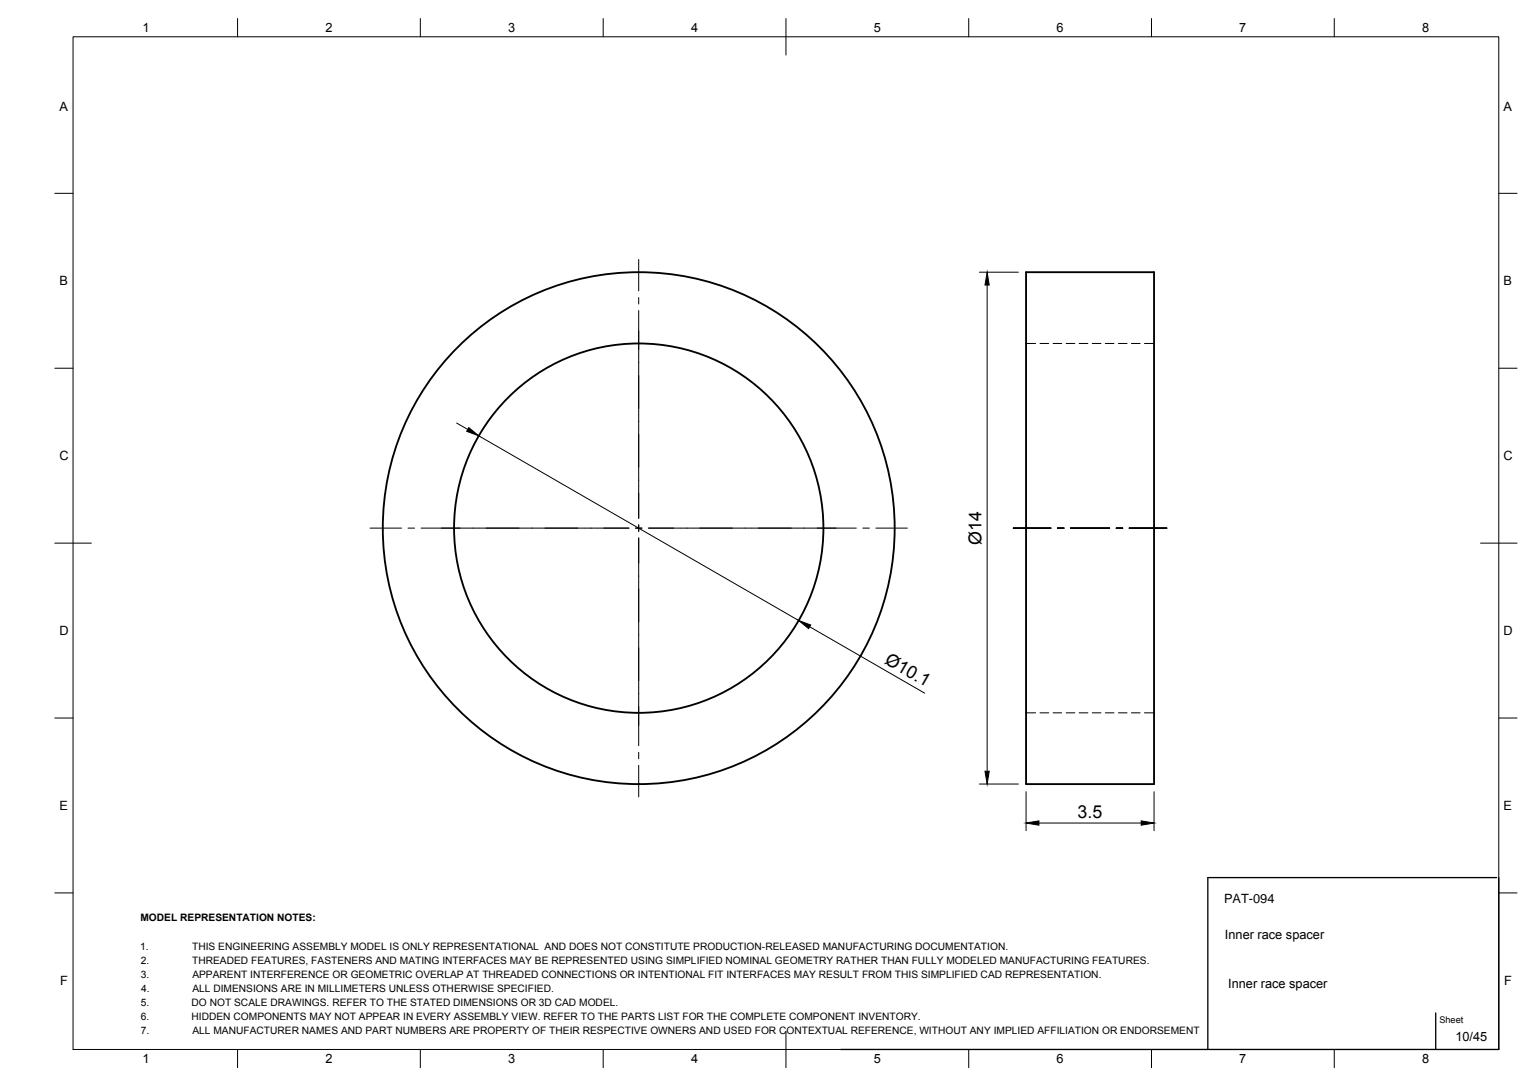
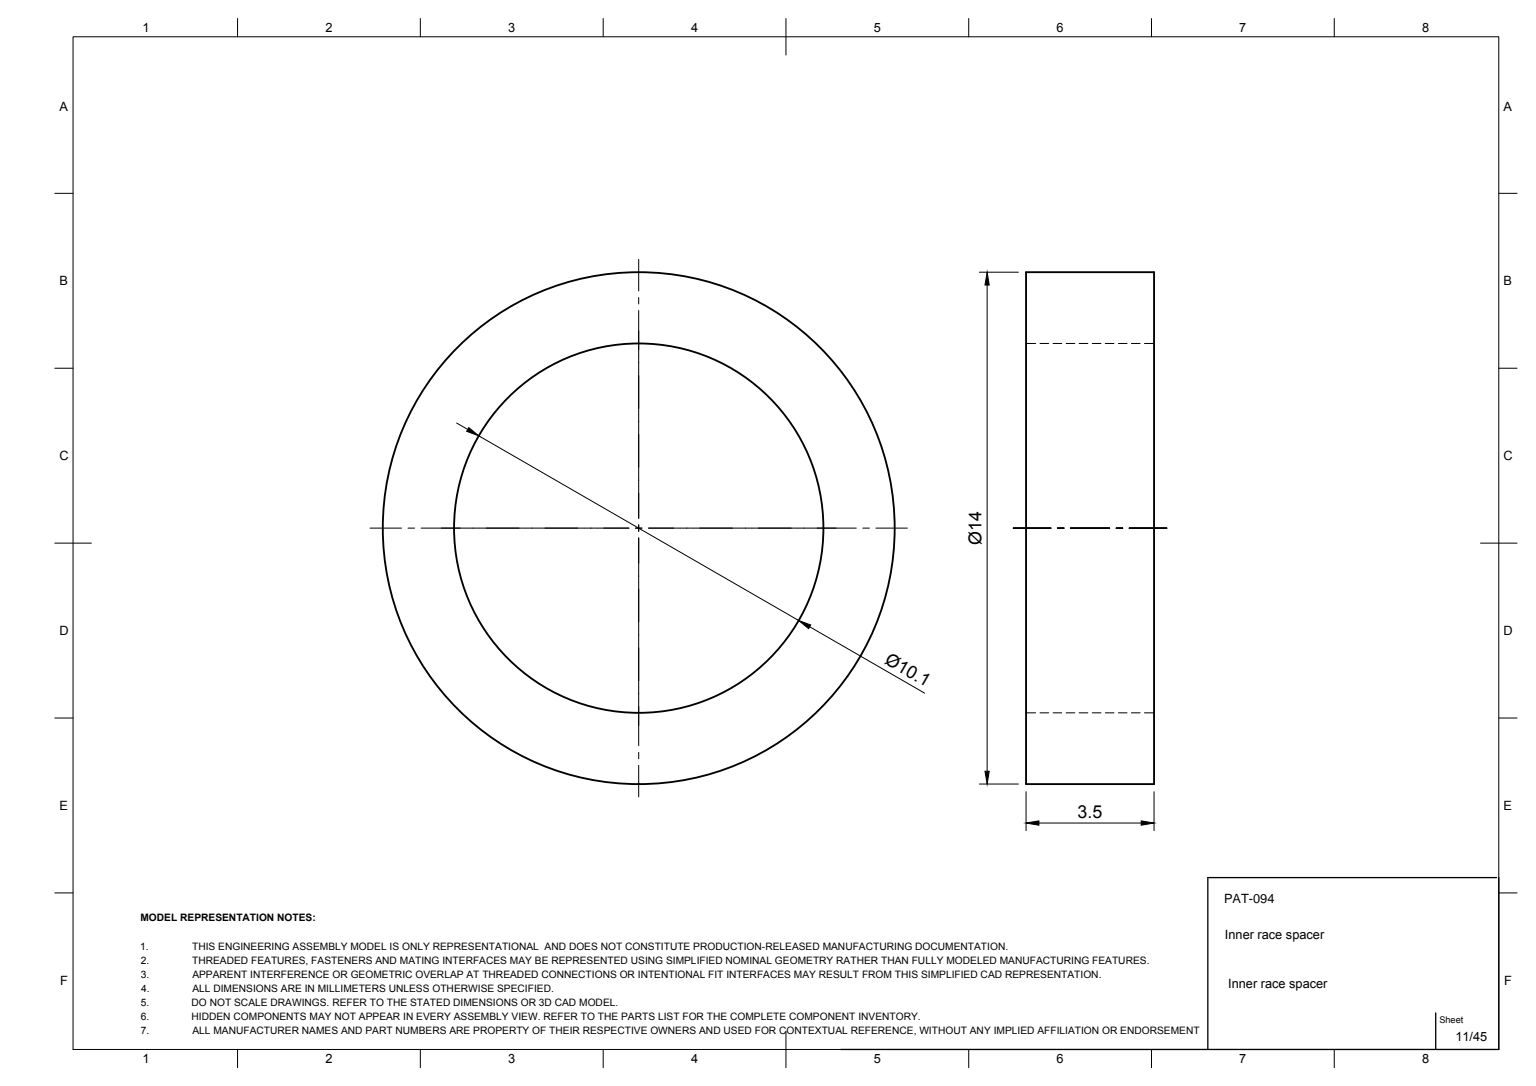
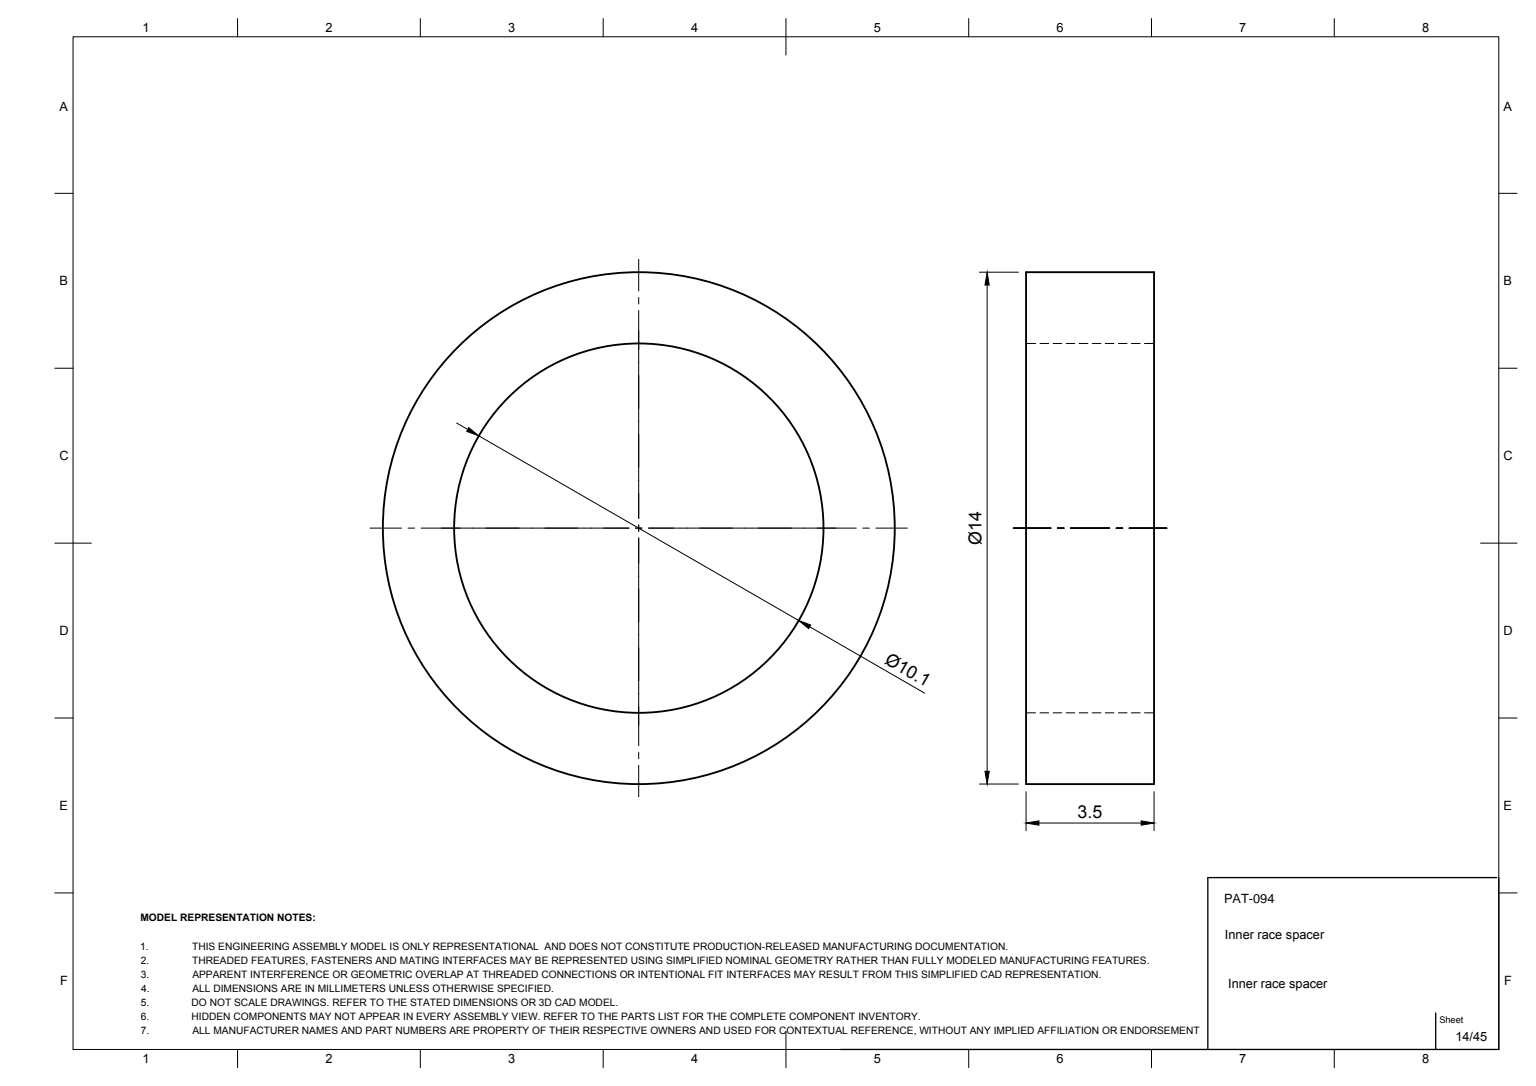
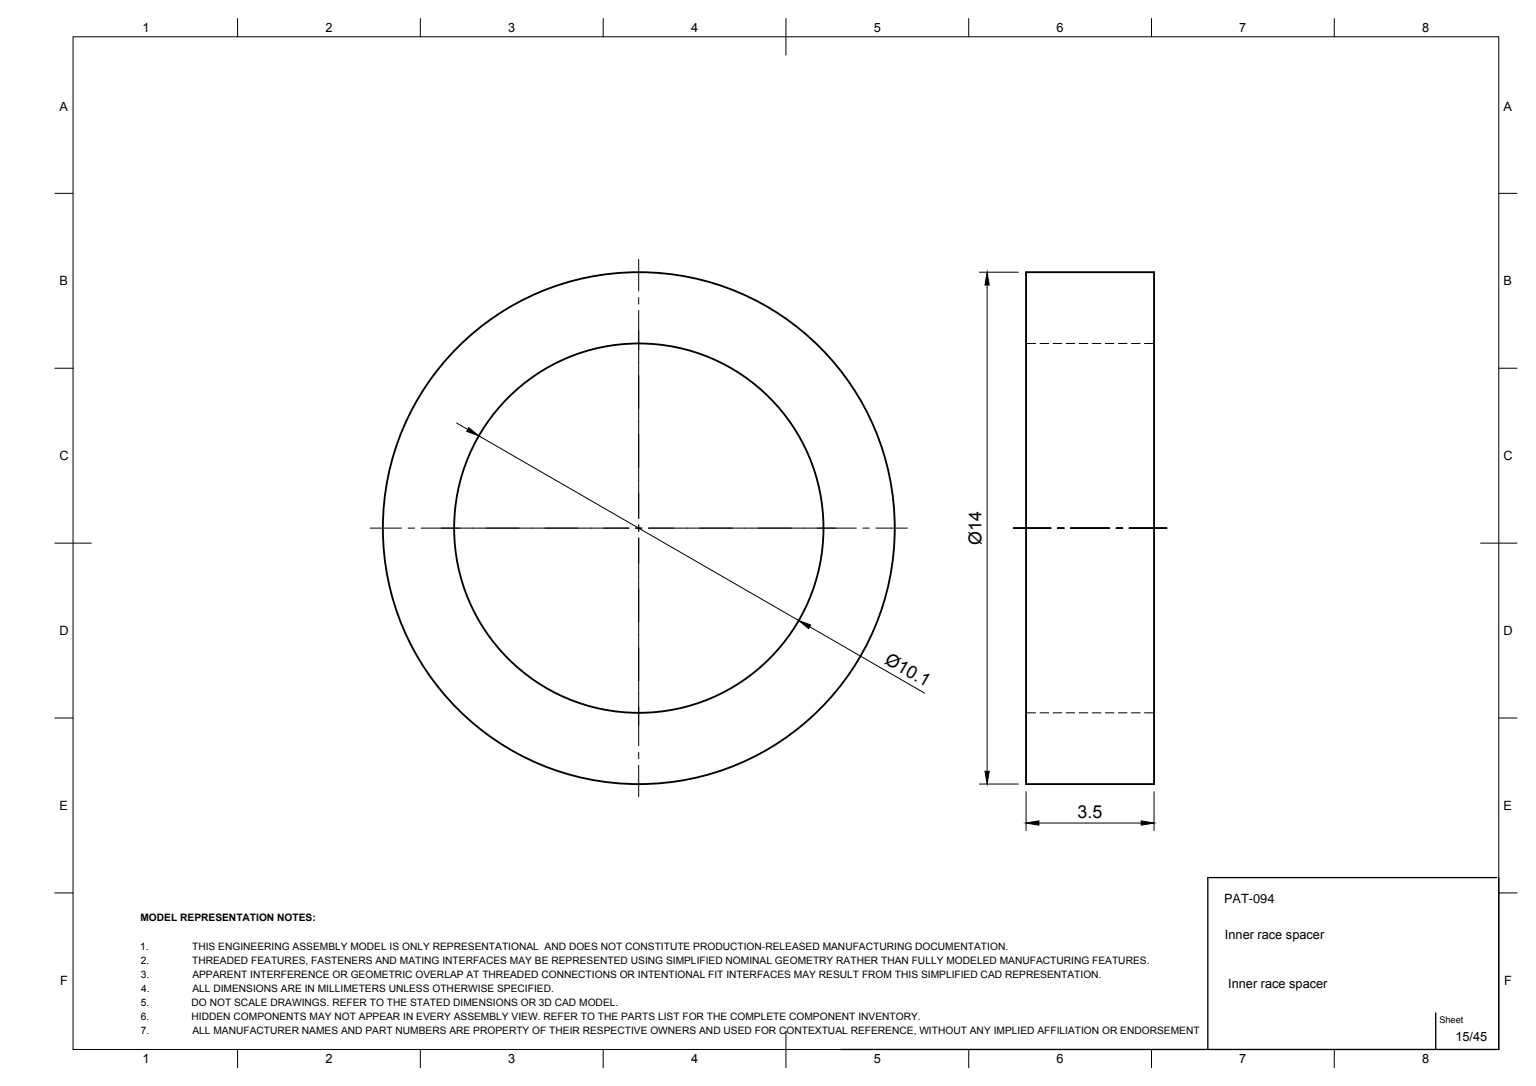
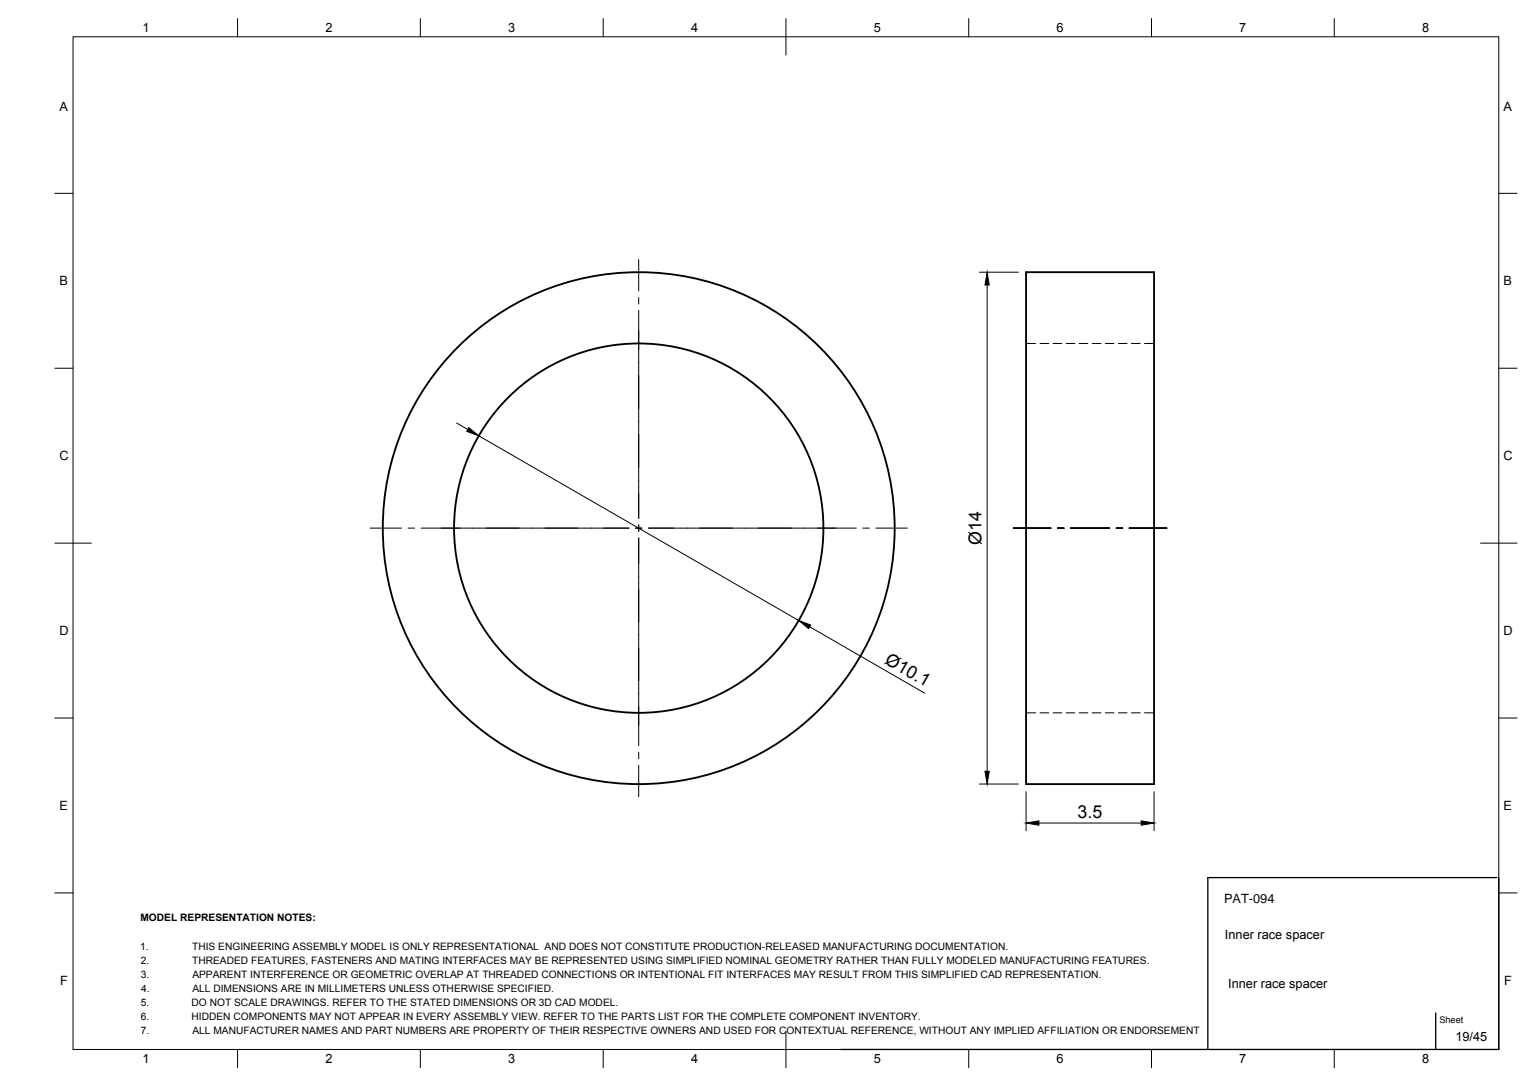
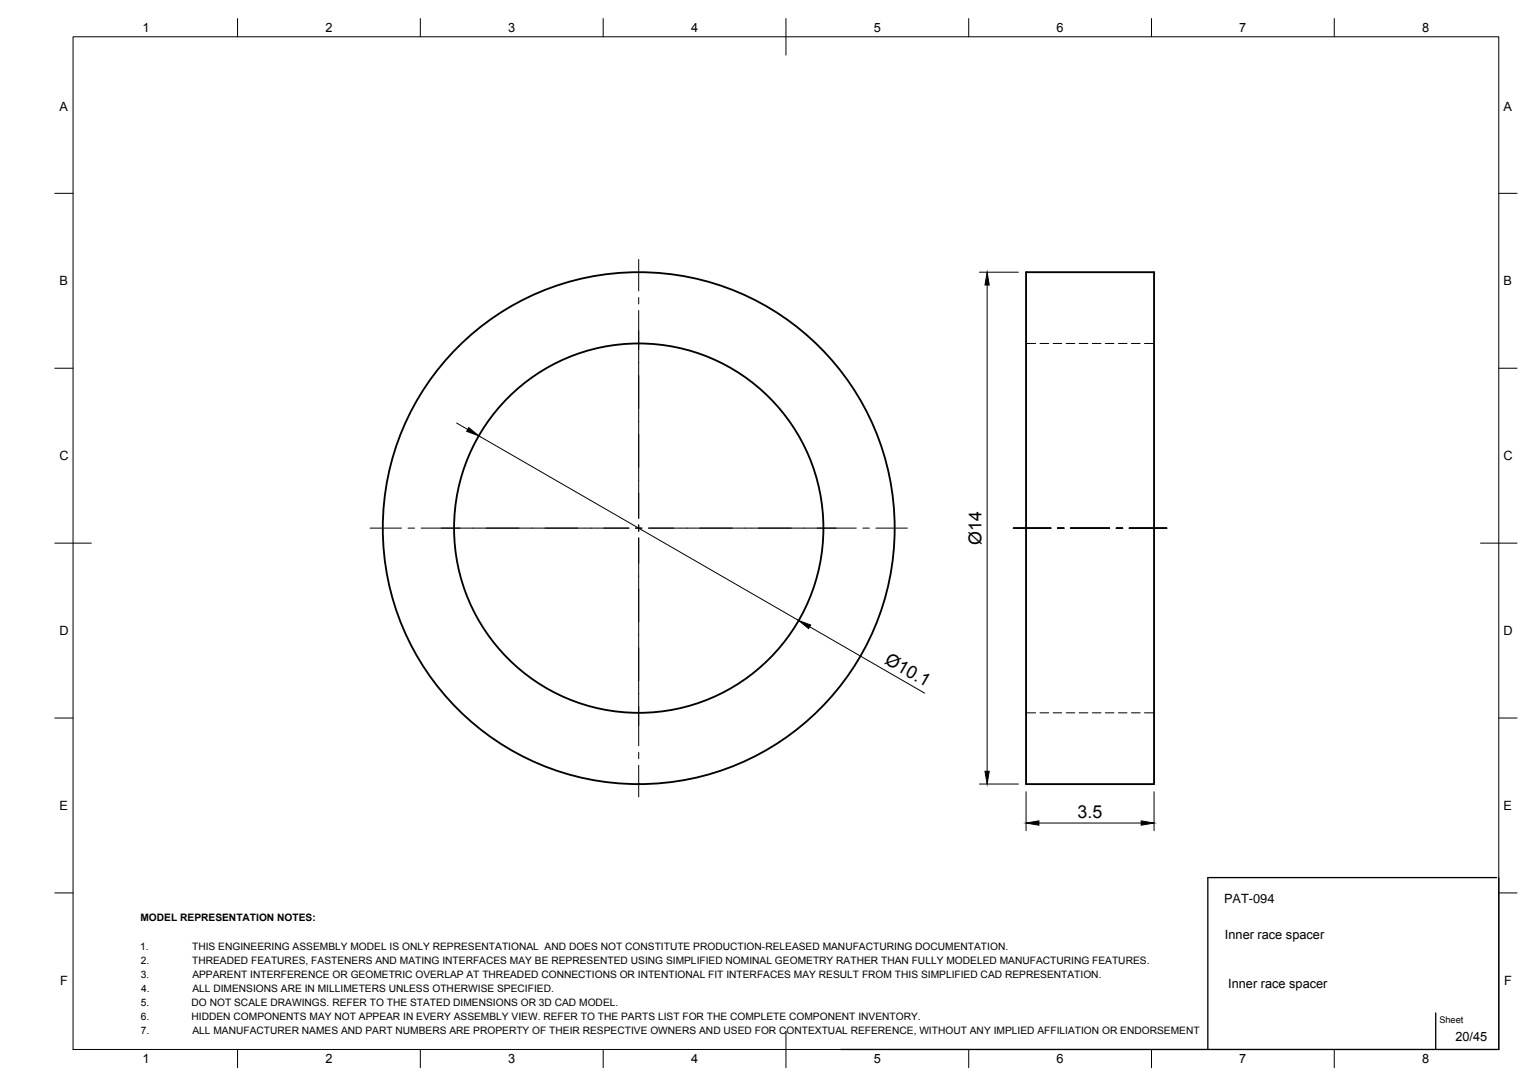
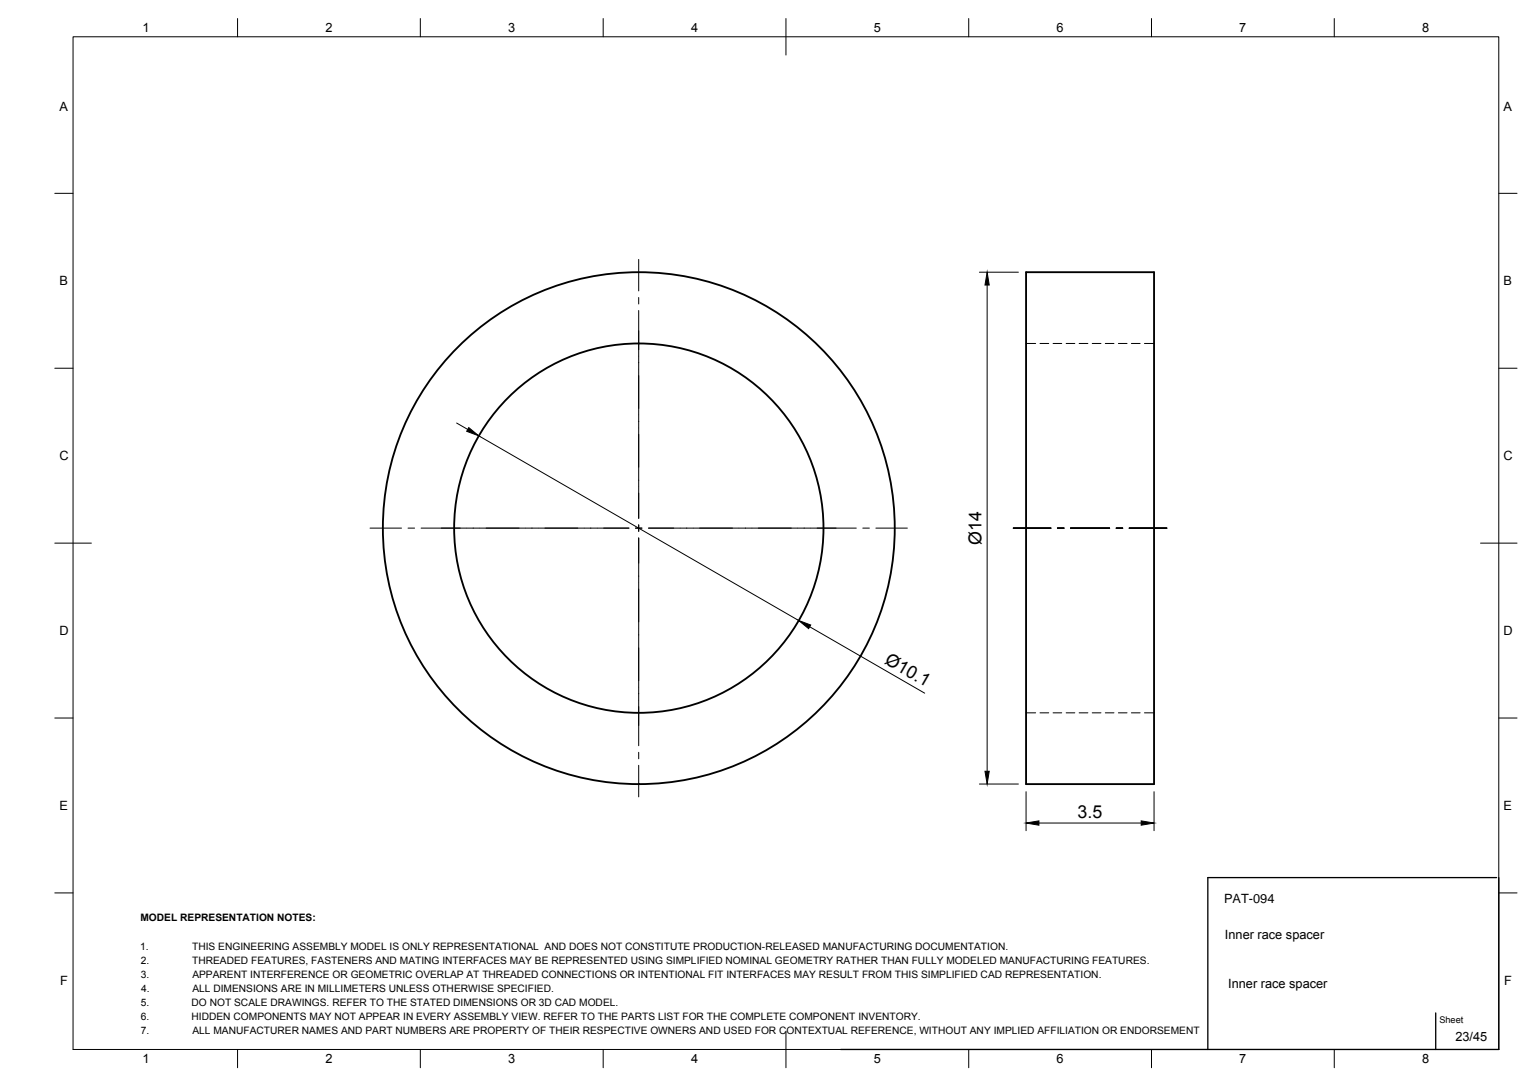
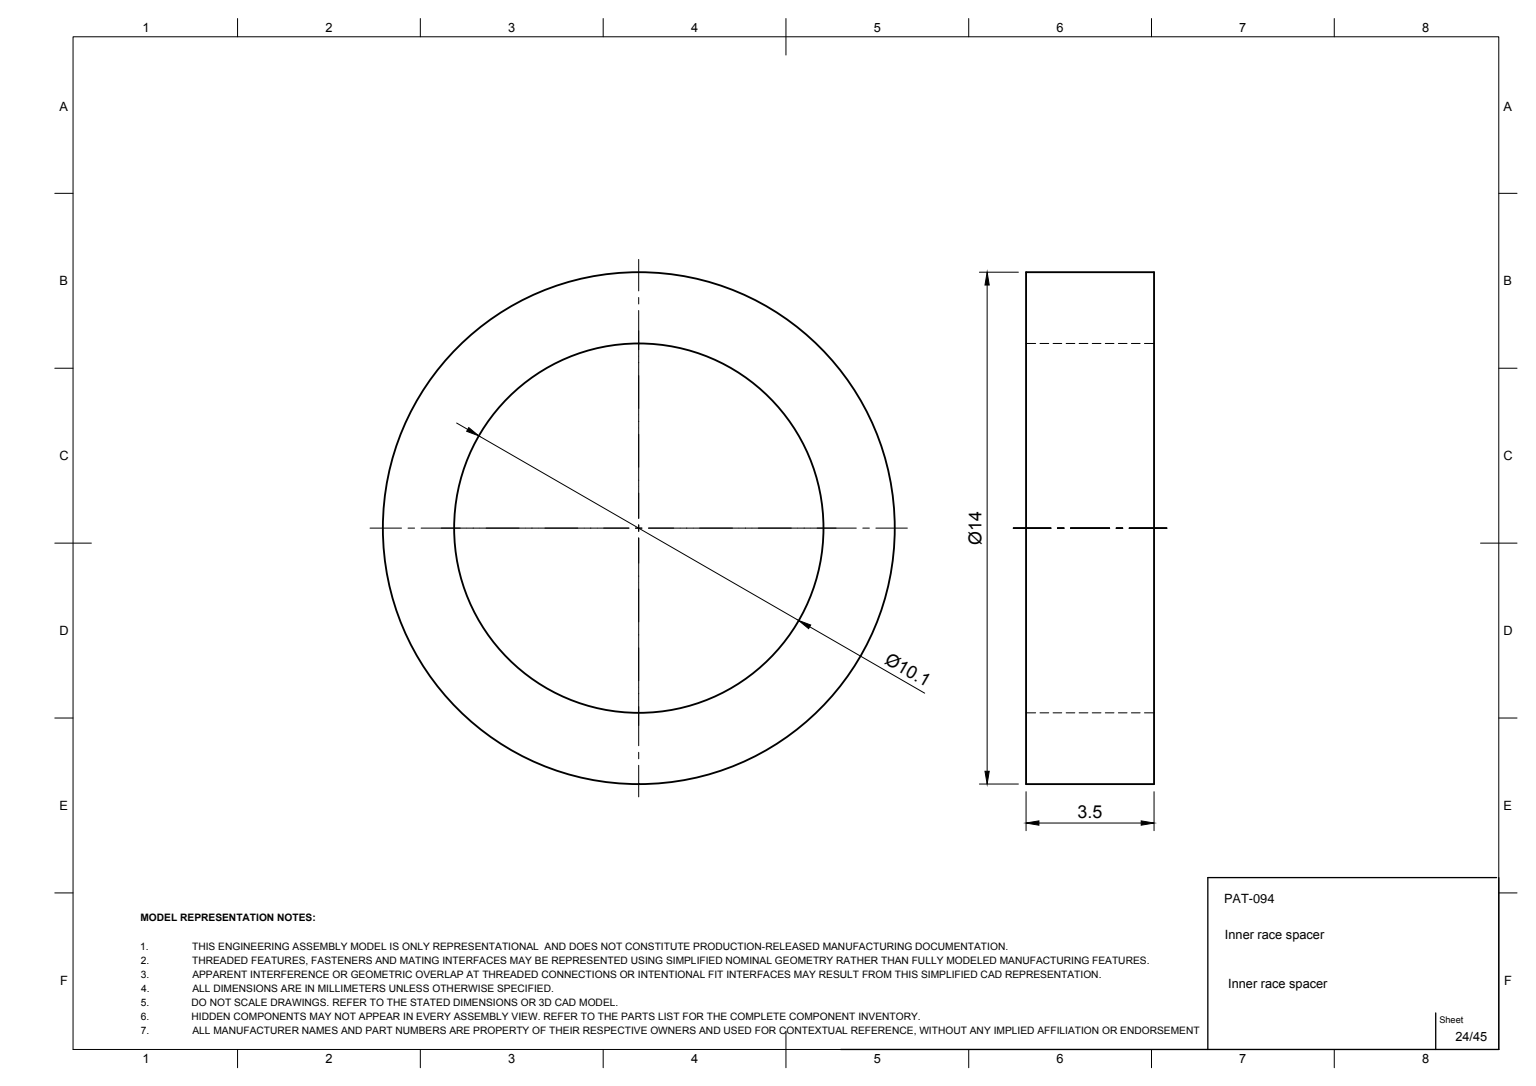
ISO-10303-21;
HEADER;
/* Generated by software containing ST-Developer
 * from STEP Tools, Inc. (www.steptools.com) 
 */

FILE_DESCRIPTION(
/* description */ ('Shaft runout checking stand'),
/* implementation_level */ '2;1');

FILE_NAME(
/* name */ 'Inner race spacer.step',
/* time_stamp */ '2026-11-02T21:12:33-08:00',
/* author */ (''),
/* organization */ (''),
/* preprocessor_version */ 'ST-DEVELOPER v20.2',
/* originating_system */ 'Autodesk Translation Framework v15.17.0.0',
/* authorisation */ '');

FILE_SCHEMA (('AUTOMOTIVE_DESIGN { 1 0 10303 214 3 1 1 }'));
ENDSEC;

DATA;
#10=MECHANICAL_DESIGN_GEOMETRIC_PRESENTATION_REPRESENTATION('',(#471),#11748);
#385=SHAPE_REPRESENTATION_RELATIONSHIP('SRR','None',#11934,#428);
#428=ADVANCED_BREP_SHAPE_REPRESENTATION('',(#522),#11710);
#471=STYLED_ITEM('',(#12170),#522);
#522=MANIFOLD_SOLID_BREP('Body1',#6214);
#601=FACE_BOUND('',#1565,.T.);
#602=FACE_BOUND('',#1567,.T.);
#724=CIRCLE('',#6916,0.505);
#725=CIRCLE('',#6917,0.505);
#726=CIRCLE('',#6919,0.7);
#727=CIRCLE('',#6920,0.7);
#962=CYLINDRICAL_SURFACE('',#6915,0.505);
#963=CYLINDRICAL_SURFACE('',#6918,0.7);
#1155=FACE_OUTER_BOUND('',#1562,.T.);
#1156=FACE_OUTER_BOUND('',#1563,.T.);
#1157=FACE_OUTER_BOUND('',#1564,.T.);
#1158=FACE_OUTER_BOUND('',#1566,.T.);
#1562=EDGE_LOOP('',(#4686,#4687,#4688,#4689));
#1563=EDGE_LOOP('',(#4690,#4691,#4692,#4693));
#1564=EDGE_LOOP('',(#4694));
#1565=EDGE_LOOP('',(#4695));
#1566=EDGE_LOOP('',(#4696));
#1567=EDGE_LOOP('',(#4697));
#2131=LINE('',#10105,#2598);
#2132=LINE('',#10111,#2599);
#2598=VECTOR('',#8104,0.505);
#2599=VECTOR('',#8111,0.7);
#3018=VERTEX_POINT('',#10102);
#3019=VERTEX_POINT('',#10104);
#3020=VERTEX_POINT('',#10108);
#3021=VERTEX_POINT('',#10110);
#3629=EDGE_CURVE('',#3018,#3018,#724,.T.);
#3630=EDGE_CURVE('',#3018,#3019,#2131,.T.);
#3631=EDGE_CURVE('',#3019,#3019,#725,.T.);
#3632=EDGE_CURVE('',#3020,#3020,#726,.T.);
#3633=EDGE_CURVE('',#3020,#3021,#2132,.T.);
#3634=EDGE_CURVE('',#3021,#3021,#727,.T.);
#4686=ORIENTED_EDGE('',*,*,#3629,.F.);
#4687=ORIENTED_EDGE('',*,*,#3630,.T.);
#4688=ORIENTED_EDGE('',*,*,#3631,.T.);
#4689=ORIENTED_EDGE('',*,*,#3630,.F.);
#4690=ORIENTED_EDGE('',*,*,#3632,.F.);
#4691=ORIENTED_EDGE('',*,*,#3633,.T.);
#4692=ORIENTED_EDGE('',*,*,#3634,.T.);
#4693=ORIENTED_EDGE('',*,*,#3633,.F.);
#4694=ORIENTED_EDGE('',*,*,#3632,.T.);
#4695=ORIENTED_EDGE('',*,*,#3629,.T.);
#4696=ORIENTED_EDGE('',*,*,#3634,.F.);
#4697=ORIENTED_EDGE('',*,*,#3631,.F.);
#5696=PLANE('',#6921);
#5697=PLANE('',#6922);
#5955=ADVANCED_FACE('',(#1155),#962,.F.);
#5956=ADVANCED_FACE('',(#1156),#963,.T.);
#5957=ADVANCED_FACE('',(#1157,#601),#5696,.T.);
#5958=ADVANCED_FACE('',(#1158,#602),#5697,.F.);
#6214=CLOSED_SHELL('',(#5955,#5956,#5957,#5958));
#6914=AXIS2_PLACEMENT_3D('',#10100,#8098,#8099);
#6915=AXIS2_PLACEMENT_3D('',#10101,#8100,#8101);
#6916=AXIS2_PLACEMENT_3D('',#10103,#8102,#8103);
#6917=AXIS2_PLACEMENT_3D('',#10106,#8105,#8106);
#6918=AXIS2_PLACEMENT_3D('',#10107,#8107,#8108);
#6919=AXIS2_PLACEMENT_3D('',#10109,#8109,#8110);
#6920=AXIS2_PLACEMENT_3D('',#10112,#8112,#8113);
#6921=AXIS2_PLACEMENT_3D('',#10113,#8114,#8115);
#6922=AXIS2_PLACEMENT_3D('',#10114,#8116,#8117);
#8098=DIRECTION('axis',(0.,0.,1.));
#8099=DIRECTION('refdir',(1.,0.,0.));
#8100=DIRECTION('center_axis',(0.,1.,0.));
#8101=DIRECTION('ref_axis',(1.,0.,0.));
#8102=DIRECTION('center_axis',(0.,-1.,0.));
#8103=DIRECTION('ref_axis',(1.,0.,0.));
#8104=DIRECTION('',(0.,-1.,0.));
#8105=DIRECTION('center_axis',(0.,-1.,0.));
#8106=DIRECTION('ref_axis',(1.,0.,0.));
#8107=DIRECTION('center_axis',(0.,1.,0.));
#8108=DIRECTION('ref_axis',(1.,0.,0.));
#8109=DIRECTION('center_axis',(0.,1.,0.));
#8110=DIRECTION('ref_axis',(1.,0.,0.));
#8111=DIRECTION('',(0.,-1.,0.));
#8112=DIRECTION('center_axis',(0.,1.,0.));
#8113=DIRECTION('ref_axis',(1.,0.,0.));
#8114=DIRECTION('center_axis',(0.,1.,0.));
#8115=DIRECTION('ref_axis',(1.,0.,0.));
#8116=DIRECTION('center_axis',(0.,1.,0.));
#8117=DIRECTION('ref_axis',(1.,0.,0.));
#10100=CARTESIAN_POINT('',(0.,0.,0.));
#10101=CARTESIAN_POINT('Origin',(-2.,-10.8,5.));
#10102=CARTESIAN_POINT('',(-2.505,-10.45,5.));
#10103=CARTESIAN_POINT('Origin',(-2.,-10.45,5.));
#10104=CARTESIAN_POINT('',(-2.505,-10.8,5.));
#10105=CARTESIAN_POINT('',(-2.505,-10.8,5.));
#10106=CARTESIAN_POINT('Origin',(-2.,-10.8,5.));
#10107=CARTESIAN_POINT('Origin',(-2.,-10.8,5.));
#10108=CARTESIAN_POINT('',(-2.7,-10.45,5.));
#10109=CARTESIAN_POINT('Origin',(-2.,-10.45,5.));
#10110=CARTESIAN_POINT('',(-2.7,-10.8,5.));
#10111=CARTESIAN_POINT('',(-2.7,-10.8,5.));
#10112=CARTESIAN_POINT('Origin',(-2.,-10.8,5.));
#10113=CARTESIAN_POINT('Origin',(-2.,-10.45,5.));
#10114=CARTESIAN_POINT('Origin',(-2.,-10.8,5.));
#11661=UNCERTAINTY_MEASURE_WITH_UNIT(LENGTH_MEASURE(0.001),#11749,
'DISTANCE_ACCURACY_VALUE',
'Maximum model space distance between geometric entities at asserted c
onnectivities');
#11699=UNCERTAINTY_MEASURE_WITH_UNIT(LENGTH_MEASURE(0.001),#11749,
'DISTANCE_ACCURACY_VALUE',
'Maximum model space distance between geometric entities at asserted c
onnectivities');
#11710=(
GEOMETRIC_REPRESENTATION_CONTEXT(3)
GLOBAL_UNCERTAINTY_ASSIGNED_CONTEXT((#11661))
GLOBAL_UNIT_ASSIGNED_CONTEXT((#11749,#11751,#11752))
REPRESENTATION_CONTEXT('','3D')
);
#11748=(
GEOMETRIC_REPRESENTATION_CONTEXT(3)
GLOBAL_UNCERTAINTY_ASSIGNED_CONTEXT((#11699))
GLOBAL_UNIT_ASSIGNED_CONTEXT((#11749,#11751,#11752))
REPRESENTATION_CONTEXT('','3D')
);
#11749=(
LENGTH_UNIT()
NAMED_UNIT(*)
SI_UNIT(.CENTI.,.METRE.)
);
#11751=(
NAMED_UNIT(*)
PLANE_ANGLE_UNIT()
SI_UNIT($,.RADIAN.)
);
#11752=(
NAMED_UNIT(*)
SI_UNIT($,.STERADIAN.)
SOLID_ANGLE_UNIT()
);
#11763=SHAPE_DEFINITION_REPRESENTATION(#11811,#11934);
#11811=PRODUCT_DEFINITION_SHAPE('',$,#11983);
#11934=SHAPE_REPRESENTATION('',(#6914),#11710);
#11972=PRODUCT_DEFINITION_CONTEXT('part definition',#12118,'design');
#11983=PRODUCT_DEFINITION('Inner race spacer','Inner race spacer',#12031,
#11972);
#12031=PRODUCT_DEFINITION_FORMATION('',$,#12130);
#12118=APPLICATION_CONTEXT(
'Core Data for Automotive Mechanical Design Process');
#12119=PRODUCT_CONTEXT('part definition',#12118,'mechanical');
#12130=PRODUCT('Inner race spacer','Inner race spacer',
'Inner race spacer',(#12119));
#12170=PRESENTATION_STYLE_ASSIGNMENT((#12175));
#12175=SURFACE_STYLE_USAGE(.BOTH.,#12180);
#12180=SURFACE_SIDE_STYLE('',(#12185));
#12185=SURFACE_STYLE_FILL_AREA(#12190);
#12190=FILL_AREA_STYLE('CAD Library Painted - Steel gray',(#12195));
#12195=FILL_AREA_STYLE_COLOUR('CAD Library Painted - Steel gray',#12200);
#12200=COLOUR_RGB('CAD Library Painted - Steel gray',0.592156862745098,
0.631372549019608,0.67843137254902);
ENDSEC;
END-ISO-10303-21;
